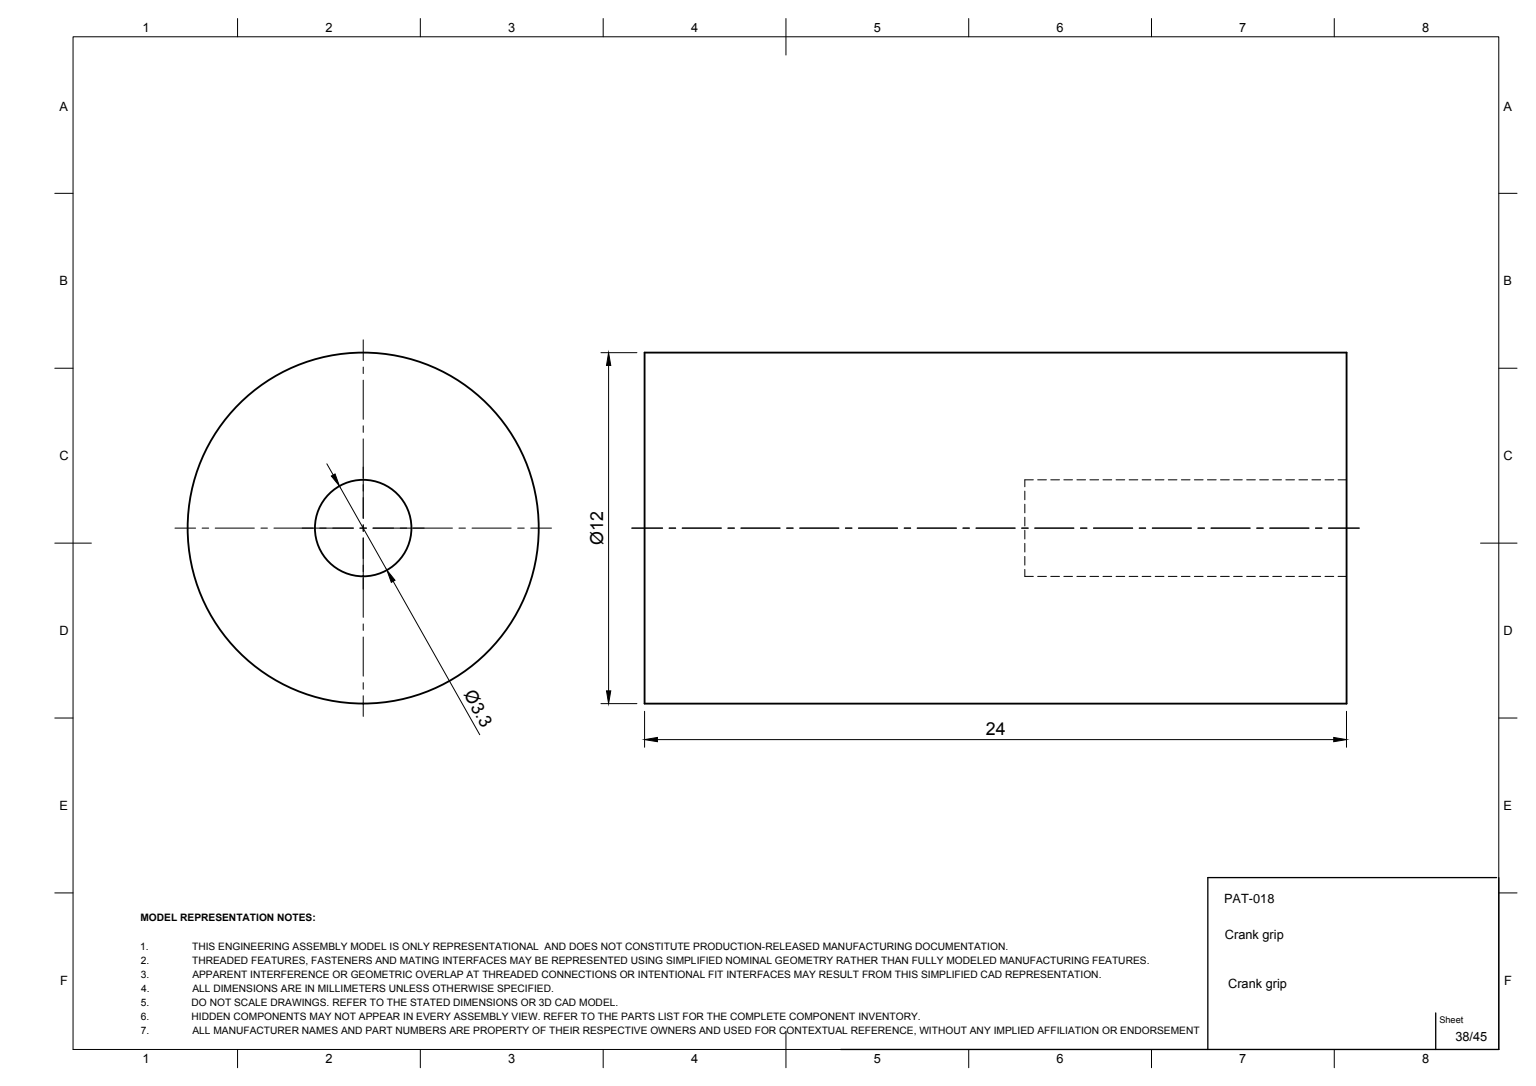
ISO-10303-21;
HEADER;
/* Generated by software containing ST-Developer
 * from STEP Tools, Inc. (www.steptools.com) 
 */

FILE_DESCRIPTION(
/* description */ ('Cam-driven reciprocating slide'),
/* implementation_level */ '2;1');

FILE_NAME(
/* name */ 'Crank grip.step',
/* time_stamp */ '2026-10-28T03:25:20-07:00',
/* author */ (''),
/* organization */ (''),
/* preprocessor_version */ 'ST-DEVELOPER v20.2',
/* originating_system */ 'Autodesk Translation Framework v15.17.0.0',
/* authorisation */ '');

FILE_SCHEMA (('AUTOMOTIVE_DESIGN { 1 0 10303 214 3 1 1 }'));
ENDSEC;

DATA;
#10=MECHANICAL_DESIGN_GEOMETRIC_PRESENTATION_REPRESENTATION('',(#458),#13277);
#377=SHAPE_REPRESENTATION_RELATIONSHIP('SRR','None',#13473,#414);
#414=ADVANCED_BREP_SHAPE_REPRESENTATION('',(#500),#13268);
#458=STYLED_ITEM('',(#13727),#500);
#500=MANIFOLD_SOLID_BREP('Body1',#6436);
#661=FACE_BOUND('',#1753,.T.);
#857=PLANE('',#7497);
#858=PLANE('',#7501);
#859=PLANE('',#7502);
#1215=FACE_OUTER_BOUND('',#1748,.T.);
#1216=FACE_OUTER_BOUND('',#1749,.T.);
#1217=FACE_OUTER_BOUND('',#1750,.T.);
#1218=FACE_OUTER_BOUND('',#1751,.T.);
#1219=FACE_OUTER_BOUND('',#1752,.T.);
#1748=EDGE_LOOP('',(#5642,#5643,#5644,#5645));
#1749=EDGE_LOOP('',(#5646));
#1750=EDGE_LOOP('',(#5647,#5648,#5649,#5650));
#1751=EDGE_LOOP('',(#5651));
#1752=EDGE_LOOP('',(#5652));
#1753=EDGE_LOOP('',(#5653));
#2185=LINE('',#12850,#2624);
#2186=LINE('',#12857,#2625);
#2624=VECTOR('',#9307,0.165);
#2625=VECTOR('',#9316,0.6);
#2997=CIRCLE('',#7495,0.165);
#2998=CIRCLE('',#7496,0.165);
#2999=CIRCLE('',#7499,0.6);
#3000=CIRCLE('',#7500,0.6);
#3476=VERTEX_POINT('',#12847);
#3477=VERTEX_POINT('',#12849);
#3478=VERTEX_POINT('',#12854);
#3479=VERTEX_POINT('',#12856);
#4211=EDGE_CURVE('',#3476,#3476,#2997,.T.);
#4212=EDGE_CURVE('',#3476,#3477,#2185,.T.);
#4213=EDGE_CURVE('',#3477,#3477,#2998,.T.);
#4214=EDGE_CURVE('',#3478,#3478,#2999,.T.);
#4215=EDGE_CURVE('',#3478,#3479,#2186,.T.);
#4216=EDGE_CURVE('',#3479,#3479,#3000,.T.);
#5642=ORIENTED_EDGE('',*,*,#4211,.F.);
#5643=ORIENTED_EDGE('',*,*,#4212,.T.);
#5644=ORIENTED_EDGE('',*,*,#4213,.T.);
#5645=ORIENTED_EDGE('',*,*,#4212,.F.);
#5646=ORIENTED_EDGE('',*,*,#4213,.F.);
#5647=ORIENTED_EDGE('',*,*,#4214,.F.);
#5648=ORIENTED_EDGE('',*,*,#4215,.T.);
#5649=ORIENTED_EDGE('',*,*,#4216,.T.);
#5650=ORIENTED_EDGE('',*,*,#4215,.F.);
#5651=ORIENTED_EDGE('',*,*,#4214,.T.);
#5652=ORIENTED_EDGE('',*,*,#4216,.F.);
#5653=ORIENTED_EDGE('',*,*,#4211,.T.);
#6002=CYLINDRICAL_SURFACE('',#7494,0.165);
#6003=CYLINDRICAL_SURFACE('',#7498,0.6);
#6333=ADVANCED_FACE('',(#1215),#6002,.F.);
#6334=ADVANCED_FACE('',(#1216),#857,.F.);
#6335=ADVANCED_FACE('',(#1217),#6003,.T.);
#6336=ADVANCED_FACE('',(#1218),#858,.T.);
#6337=ADVANCED_FACE('',(#1219,#661),#859,.F.);
#6436=CLOSED_SHELL('',(#6333,#6334,#6335,#6336,#6337));
#7493=AXIS2_PLACEMENT_3D('',#12845,#9301,#9302);
#7494=AXIS2_PLACEMENT_3D('',#12846,#9303,#9304);
#7495=AXIS2_PLACEMENT_3D('',#12848,#9305,#9306);
#7496=AXIS2_PLACEMENT_3D('',#12851,#9308,#9309);
#7497=AXIS2_PLACEMENT_3D('',#12852,#9310,#9311);
#7498=AXIS2_PLACEMENT_3D('',#12853,#9312,#9313);
#7499=AXIS2_PLACEMENT_3D('',#12855,#9314,#9315);
#7500=AXIS2_PLACEMENT_3D('',#12858,#9317,#9318);
#7501=AXIS2_PLACEMENT_3D('',#12859,#9319,#9320);
#7502=AXIS2_PLACEMENT_3D('',#12860,#9321,#9322);
#9301=DIRECTION('axis',(0.,0.,1.));
#9302=DIRECTION('refdir',(1.,0.,0.));
#9303=DIRECTION('center_axis',(0.,1.,0.));
#9304=DIRECTION('ref_axis',(1.,0.,0.));
#9305=DIRECTION('center_axis',(0.,1.,0.));
#9306=DIRECTION('ref_axis',(1.,0.,0.));
#9307=DIRECTION('',(0.,1.,0.));
#9308=DIRECTION('center_axis',(0.,1.,0.));
#9309=DIRECTION('ref_axis',(1.,0.,0.));
#9310=DIRECTION('center_axis',(0.,1.,0.));
#9311=DIRECTION('ref_axis',(1.,0.,0.));
#9312=DIRECTION('center_axis',(0.,1.,0.));
#9313=DIRECTION('ref_axis',(1.,0.,0.));
#9314=DIRECTION('center_axis',(0.,1.,0.));
#9315=DIRECTION('ref_axis',(1.,0.,0.));
#9316=DIRECTION('',(0.,-1.,0.));
#9317=DIRECTION('center_axis',(0.,1.,0.));
#9318=DIRECTION('ref_axis',(1.,0.,0.));
#9319=DIRECTION('center_axis',(0.,1.,0.));
#9320=DIRECTION('ref_axis',(1.,0.,0.));
#9321=DIRECTION('center_axis',(0.,1.,0.));
#9322=DIRECTION('ref_axis',(1.,0.,0.));
#12845=CARTESIAN_POINT('',(0.,0.,0.));
#12846=CARTESIAN_POINT('Origin',(2.5,5.7,4.));
#12847=CARTESIAN_POINT('',(2.335,5.8,4.));
#12848=CARTESIAN_POINT('Origin',(2.5,5.8,4.));
#12849=CARTESIAN_POINT('',(2.335,6.9,4.));
#12850=CARTESIAN_POINT('',(2.335,5.7,4.));
#12851=CARTESIAN_POINT('Origin',(2.5,6.9,4.));
#12852=CARTESIAN_POINT('Origin',(2.5,6.9,4.));
#12853=CARTESIAN_POINT('Origin',(2.5,5.8,4.));
#12854=CARTESIAN_POINT('',(1.9,8.2,4.));
#12855=CARTESIAN_POINT('Origin',(2.5,8.2,4.));
#12856=CARTESIAN_POINT('',(1.9,5.8,4.));
#12857=CARTESIAN_POINT('',(1.9,5.8,4.));
#12858=CARTESIAN_POINT('Origin',(2.5,5.8,4.));
#12859=CARTESIAN_POINT('Origin',(2.5,8.2,4.));
#12860=CARTESIAN_POINT('Origin',(2.5,5.8,4.));
#13224=UNCERTAINTY_MEASURE_WITH_UNIT(LENGTH_MEASURE(0.001),#13278,
'DISTANCE_ACCURACY_VALUE',
'Maximum model space distance between geometric entities at asserted c
onnectivities');
#13233=UNCERTAINTY_MEASURE_WITH_UNIT(LENGTH_MEASURE(0.001),#13278,
'DISTANCE_ACCURACY_VALUE',
'Maximum model space distance between geometric entities at asserted c
onnectivities');
#13268=(
GEOMETRIC_REPRESENTATION_CONTEXT(3)
GLOBAL_UNCERTAINTY_ASSIGNED_CONTEXT((#13224))
GLOBAL_UNIT_ASSIGNED_CONTEXT((#13278,#13280,#13281))
REPRESENTATION_CONTEXT('','3D')
);
#13277=(
GEOMETRIC_REPRESENTATION_CONTEXT(3)
GLOBAL_UNCERTAINTY_ASSIGNED_CONTEXT((#13233))
GLOBAL_UNIT_ASSIGNED_CONTEXT((#13278,#13280,#13281))
REPRESENTATION_CONTEXT('','3D')
);
#13278=(
LENGTH_UNIT()
NAMED_UNIT(*)
SI_UNIT(.CENTI.,.METRE.)
);
#13280=(
NAMED_UNIT(*)
PLANE_ANGLE_UNIT()
SI_UNIT($,.RADIAN.)
);
#13281=(
NAMED_UNIT(*)
SI_UNIT($,.STERADIAN.)
SOLID_ANGLE_UNIT()
);
#13316=SHAPE_DEFINITION_REPRESENTATION(#13366,#13473);
#13366=PRODUCT_DEFINITION_SHAPE('',$,#13517);
#13473=SHAPE_REPRESENTATION('',(#7493),#13268);
#13482=PRODUCT_DEFINITION_CONTEXT('part definition',#13613,'design');
#13517=PRODUCT_DEFINITION('Crank grip','Crank grip',#13560,#13482);
#13560=PRODUCT_DEFINITION_FORMATION('',$,#13649);
#13613=APPLICATION_CONTEXT(
'Core Data for Automotive Mechanical Design Process');
#13614=PRODUCT_CONTEXT('part definition',#13613,'mechanical');
#13649=PRODUCT('Crank grip','Crank grip','Crank grip',(#13614));
#13721=COLOUR_RGB('Black',0.12,0.14,0.17);
#13722=FILL_AREA_STYLE_COLOUR('',#13721);
#13723=FILL_AREA_STYLE('',(#13722));
#13724=SURFACE_STYLE_FILL_AREA(#13723);
#13725=SURFACE_SIDE_STYLE('',(#13724));
#13726=SURFACE_STYLE_USAGE(.BOTH.,#13725);
#13727=PRESENTATION_STYLE_ASSIGNMENT((#13726));
ENDSEC;
END-ISO-10303-21;
